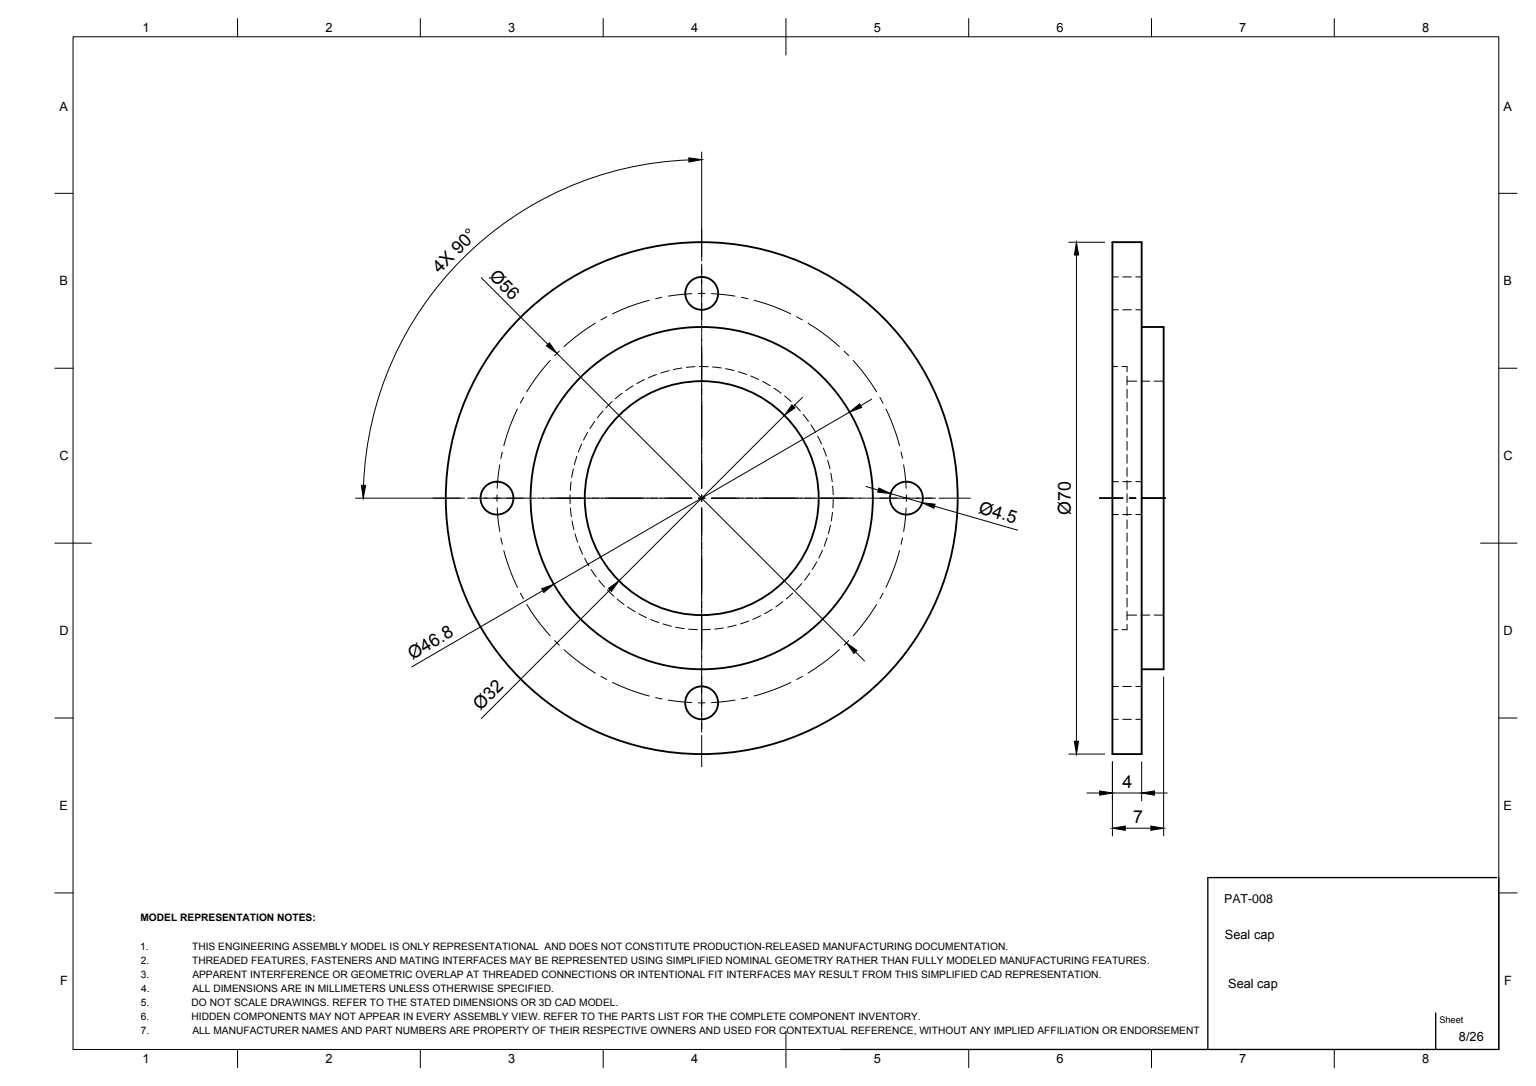
ISO-10303-21;
HEADER;
/* Generated by software containing ST-Developer
 * from STEP Tools, Inc. (www.steptools.com) 
 */

FILE_DESCRIPTION(
/* description */ ('Bearing housing with oil seal and end cap'),
/* implementation_level */ '2;1');

FILE_NAME(
/* name */ 'Seal cap.step',
/* time_stamp */ '2026-10-28T03:23:10-07:00',
/* author */ (''),
/* organization */ (''),
/* preprocessor_version */ 'ST-DEVELOPER v20.2',
/* originating_system */ 'Autodesk Translation Framework v15.17.0.0',
/* authorisation */ '');

FILE_SCHEMA (('AUTOMOTIVE_DESIGN { 1 0 10303 214 3 1 1 }'));
ENDSEC;

DATA;
#10=MECHANICAL_DESIGN_GEOMETRIC_PRESENTATION_REPRESENTATION('',(#262),#7871);
#220=SHAPE_REPRESENTATION_RELATIONSHIP('SRR','None',#7967,#241);
#241=ADVANCED_BREP_SHAPE_REPRESENTATION('',(#291),#7851);
#262=STYLED_ITEM('',(#8160),#291);
#291=MANIFOLD_SOLID_BREP('Body1',#4088);
#345=FACE_BOUND('',#895,.T.);
#346=FACE_BOUND('',#898,.T.);
#347=FACE_BOUND('',#902,.T.);
#348=FACE_BOUND('',#903,.T.);
#349=FACE_BOUND('',#904,.T.);
#350=FACE_BOUND('',#905,.T.);
#351=FACE_BOUND('',#906,.T.);
#352=FACE_BOUND('',#908,.T.);
#353=FACE_BOUND('',#909,.T.);
#354=FACE_BOUND('',#910,.T.);
#355=FACE_BOUND('',#911,.T.);
#356=FACE_BOUND('',#912,.T.);
#444=PLANE('',#4473);
#445=PLANE('',#4478);
#446=PLANE('',#4484);
#447=PLANE('',#4485);
#608=FACE_OUTER_BOUND('',#889,.T.);
#609=FACE_OUTER_BOUND('',#890,.T.);
#610=FACE_OUTER_BOUND('',#891,.T.);
#611=FACE_OUTER_BOUND('',#892,.T.);
#612=FACE_OUTER_BOUND('',#893,.T.);
#613=FACE_OUTER_BOUND('',#894,.T.);
#614=FACE_OUTER_BOUND('',#896,.T.);
#615=FACE_OUTER_BOUND('',#897,.T.);
#616=FACE_OUTER_BOUND('',#899,.T.);
#617=FACE_OUTER_BOUND('',#900,.T.);
#618=FACE_OUTER_BOUND('',#901,.T.);
#619=FACE_OUTER_BOUND('',#907,.T.);
#889=EDGE_LOOP('',(#2975,#2976,#2977,#2978));
#890=EDGE_LOOP('',(#2979,#2980,#2981,#2982));
#891=EDGE_LOOP('',(#2983,#2984,#2985,#2986));
#892=EDGE_LOOP('',(#2987,#2988,#2989,#2990));
#893=EDGE_LOOP('',(#2991,#2992,#2993,#2994));
#894=EDGE_LOOP('',(#2995));
#895=EDGE_LOOP('',(#2996));
#896=EDGE_LOOP('',(#2997,#2998,#2999,#3000));
#897=EDGE_LOOP('',(#3001));
#898=EDGE_LOOP('',(#3002));
#899=EDGE_LOOP('',(#3003,#3004,#3005,#3006));
#900=EDGE_LOOP('',(#3007,#3008,#3009,#3010));
#901=EDGE_LOOP('',(#3011));
#902=EDGE_LOOP('',(#3012));
#903=EDGE_LOOP('',(#3013));
#904=EDGE_LOOP('',(#3014));
#905=EDGE_LOOP('',(#3015));
#906=EDGE_LOOP('',(#3016));
#907=EDGE_LOOP('',(#3017));
#908=EDGE_LOOP('',(#3018));
#909=EDGE_LOOP('',(#3019));
#910=EDGE_LOOP('',(#3020));
#911=EDGE_LOOP('',(#3021));
#912=EDGE_LOOP('',(#3022));
#1215=LINE('',#6464,#1477);
#1216=LINE('',#6470,#1478);
#1217=LINE('',#6476,#1479);
#1218=LINE('',#6482,#1480);
#1219=LINE('',#6488,#1481);
#1220=LINE('',#6497,#1482);
#1221=LINE('',#6503,#1483);
#1222=LINE('',#6508,#1484);
#1477=VECTOR('',#5172,0.225);
#1478=VECTOR('',#5179,0.225);
#1479=VECTOR('',#5186,0.225);
#1480=VECTOR('',#5193,0.225);
#1481=VECTOR('',#5200,2.34);
#1482=VECTOR('',#5211,1.8);
#1483=VECTOR('',#5220,1.6);
#1484=VECTOR('',#5225,3.5);
#1719=CIRCLE('',#4459,0.225);
#1720=CIRCLE('',#4460,0.225);
#1721=CIRCLE('',#4462,0.225);
#1722=CIRCLE('',#4463,0.225);
#1723=CIRCLE('',#4465,0.225);
#1724=CIRCLE('',#4466,0.225);
#1725=CIRCLE('',#4468,0.225);
#1726=CIRCLE('',#4469,0.225);
#1727=CIRCLE('',#4471,2.34);
#1728=CIRCLE('',#4472,2.34);
#1729=CIRCLE('',#4474,1.6);
#1730=CIRCLE('',#4476,1.8);
#1731=CIRCLE('',#4477,1.8);
#1732=CIRCLE('',#4479,1.6);
#1733=CIRCLE('',#4482,3.5);
#1734=CIRCLE('',#4483,3.5);
#1967=VERTEX_POINT('',#6461);
#1968=VERTEX_POINT('',#6463);
#1969=VERTEX_POINT('',#6467);
#1970=VERTEX_POINT('',#6469);
#1971=VERTEX_POINT('',#6473);
#1972=VERTEX_POINT('',#6475);
#1973=VERTEX_POINT('',#6479);
#1974=VERTEX_POINT('',#6481);
#1975=VERTEX_POINT('',#6485);
#1976=VERTEX_POINT('',#6487);
#1977=VERTEX_POINT('',#6491);
#1978=VERTEX_POINT('',#6494);
#1979=VERTEX_POINT('',#6496);
#1980=VERTEX_POINT('',#6500);
#1981=VERTEX_POINT('',#6505);
#1982=VERTEX_POINT('',#6507);
#2351=EDGE_CURVE('',#1967,#1967,#1719,.T.);
#2352=EDGE_CURVE('',#1967,#1968,#1215,.T.);
#2353=EDGE_CURVE('',#1968,#1968,#1720,.T.);
#2354=EDGE_CURVE('',#1969,#1969,#1721,.T.);
#2355=EDGE_CURVE('',#1969,#1970,#1216,.T.);
#2356=EDGE_CURVE('',#1970,#1970,#1722,.T.);
#2357=EDGE_CURVE('',#1971,#1971,#1723,.T.);
#2358=EDGE_CURVE('',#1971,#1972,#1217,.T.);
#2359=EDGE_CURVE('',#1972,#1972,#1724,.T.);
#2360=EDGE_CURVE('',#1973,#1973,#1725,.T.);
#2361=EDGE_CURVE('',#1973,#1974,#1218,.T.);
#2362=EDGE_CURVE('',#1974,#1974,#1726,.T.);
#2363=EDGE_CURVE('',#1975,#1975,#1727,.T.);
#2364=EDGE_CURVE('',#1975,#1976,#1219,.T.);
#2365=EDGE_CURVE('',#1976,#1976,#1728,.T.);
#2366=EDGE_CURVE('',#1977,#1977,#1729,.T.);
#2367=EDGE_CURVE('',#1978,#1978,#1730,.T.);
#2368=EDGE_CURVE('',#1978,#1979,#1220,.T.);
#2369=EDGE_CURVE('',#1979,#1979,#1731,.T.);
#2370=EDGE_CURVE('',#1980,#1980,#1732,.T.);
#2371=EDGE_CURVE('',#1977,#1980,#1221,.T.);
#2372=EDGE_CURVE('',#1981,#1981,#1733,.T.);
#2373=EDGE_CURVE('',#1981,#1982,#1222,.T.);
#2374=EDGE_CURVE('',#1982,#1982,#1734,.T.);
#2975=ORIENTED_EDGE('',*,*,#2351,.F.);
#2976=ORIENTED_EDGE('',*,*,#2352,.T.);
#2977=ORIENTED_EDGE('',*,*,#2353,.F.);
#2978=ORIENTED_EDGE('',*,*,#2352,.F.);
#2979=ORIENTED_EDGE('',*,*,#2354,.F.);
#2980=ORIENTED_EDGE('',*,*,#2355,.T.);
#2981=ORIENTED_EDGE('',*,*,#2356,.F.);
#2982=ORIENTED_EDGE('',*,*,#2355,.F.);
#2983=ORIENTED_EDGE('',*,*,#2357,.F.);
#2984=ORIENTED_EDGE('',*,*,#2358,.T.);
#2985=ORIENTED_EDGE('',*,*,#2359,.F.);
#2986=ORIENTED_EDGE('',*,*,#2358,.F.);
#2987=ORIENTED_EDGE('',*,*,#2360,.F.);
#2988=ORIENTED_EDGE('',*,*,#2361,.T.);
#2989=ORIENTED_EDGE('',*,*,#2362,.F.);
#2990=ORIENTED_EDGE('',*,*,#2361,.F.);
#2991=ORIENTED_EDGE('',*,*,#2363,.F.);
#2992=ORIENTED_EDGE('',*,*,#2364,.T.);
#2993=ORIENTED_EDGE('',*,*,#2365,.F.);
#2994=ORIENTED_EDGE('',*,*,#2364,.F.);
#2995=ORIENTED_EDGE('',*,*,#2363,.T.);
#2996=ORIENTED_EDGE('',*,*,#2366,.T.);
#2997=ORIENTED_EDGE('',*,*,#2367,.F.);
#2998=ORIENTED_EDGE('',*,*,#2368,.T.);
#2999=ORIENTED_EDGE('',*,*,#2369,.T.);
#3000=ORIENTED_EDGE('',*,*,#2368,.F.);
#3001=ORIENTED_EDGE('',*,*,#2369,.F.);
#3002=ORIENTED_EDGE('',*,*,#2370,.F.);
#3003=ORIENTED_EDGE('',*,*,#2366,.F.);
#3004=ORIENTED_EDGE('',*,*,#2371,.T.);
#3005=ORIENTED_EDGE('',*,*,#2370,.T.);
#3006=ORIENTED_EDGE('',*,*,#2371,.F.);
#3007=ORIENTED_EDGE('',*,*,#2372,.F.);
#3008=ORIENTED_EDGE('',*,*,#2373,.T.);
#3009=ORIENTED_EDGE('',*,*,#2374,.T.);
#3010=ORIENTED_EDGE('',*,*,#2373,.F.);
#3011=ORIENTED_EDGE('',*,*,#2372,.T.);
#3012=ORIENTED_EDGE('',*,*,#2365,.T.);
#3013=ORIENTED_EDGE('',*,*,#2362,.T.);
#3014=ORIENTED_EDGE('',*,*,#2359,.T.);
#3015=ORIENTED_EDGE('',*,*,#2356,.T.);
#3016=ORIENTED_EDGE('',*,*,#2353,.T.);
#3017=ORIENTED_EDGE('',*,*,#2374,.F.);
#3018=ORIENTED_EDGE('',*,*,#2367,.T.);
#3019=ORIENTED_EDGE('',*,*,#2360,.T.);
#3020=ORIENTED_EDGE('',*,*,#2357,.T.);
#3021=ORIENTED_EDGE('',*,*,#2354,.T.);
#3022=ORIENTED_EDGE('',*,*,#2351,.T.);
#3779=CYLINDRICAL_SURFACE('',#4458,0.225);
#3780=CYLINDRICAL_SURFACE('',#4461,0.225);
#3781=CYLINDRICAL_SURFACE('',#4464,0.225);
#3782=CYLINDRICAL_SURFACE('',#4467,0.225);
#3783=CYLINDRICAL_SURFACE('',#4470,2.34);
#3784=CYLINDRICAL_SURFACE('',#4475,1.8);
#3785=CYLINDRICAL_SURFACE('',#4480,1.6);
#3786=CYLINDRICAL_SURFACE('',#4481,3.5);
#3890=ADVANCED_FACE('',(#608),#3779,.F.);
#3891=ADVANCED_FACE('',(#609),#3780,.F.);
#3892=ADVANCED_FACE('',(#610),#3781,.F.);
#3893=ADVANCED_FACE('',(#611),#3782,.F.);
#3894=ADVANCED_FACE('',(#612),#3783,.T.);
#3895=ADVANCED_FACE('',(#613,#345),#444,.T.);
#3896=ADVANCED_FACE('',(#614),#3784,.F.);
#3897=ADVANCED_FACE('',(#615,#346),#445,.F.);
#3898=ADVANCED_FACE('',(#616),#3785,.F.);
#3899=ADVANCED_FACE('',(#617),#3786,.T.);
#3900=ADVANCED_FACE('',(#618,#347,#348,#349,#350,#351),#446,.T.);
#3901=ADVANCED_FACE('',(#619,#352,#353,#354,#355,#356),#447,.F.);
#4088=CLOSED_SHELL('',(#3890,#3891,#3892,#3893,#3894,#3895,#3896,#3897,
#3898,#3899,#3900,#3901));
#4457=AXIS2_PLACEMENT_3D('',#6459,#5166,#5167);
#4458=AXIS2_PLACEMENT_3D('',#6460,#5168,#5169);
#4459=AXIS2_PLACEMENT_3D('',#6462,#5170,#5171);
#4460=AXIS2_PLACEMENT_3D('',#6465,#5173,#5174);
#4461=AXIS2_PLACEMENT_3D('',#6466,#5175,#5176);
#4462=AXIS2_PLACEMENT_3D('',#6468,#5177,#5178);
#4463=AXIS2_PLACEMENT_3D('',#6471,#5180,#5181);
#4464=AXIS2_PLACEMENT_3D('',#6472,#5182,#5183);
#4465=AXIS2_PLACEMENT_3D('',#6474,#5184,#5185);
#4466=AXIS2_PLACEMENT_3D('',#6477,#5187,#5188);
#4467=AXIS2_PLACEMENT_3D('',#6478,#5189,#5190);
#4468=AXIS2_PLACEMENT_3D('',#6480,#5191,#5192);
#4469=AXIS2_PLACEMENT_3D('',#6483,#5194,#5195);
#4470=AXIS2_PLACEMENT_3D('',#6484,#5196,#5197);
#4471=AXIS2_PLACEMENT_3D('',#6486,#5198,#5199);
#4472=AXIS2_PLACEMENT_3D('',#6489,#5201,#5202);
#4473=AXIS2_PLACEMENT_3D('',#6490,#5203,#5204);
#4474=AXIS2_PLACEMENT_3D('',#6492,#5205,#5206);
#4475=AXIS2_PLACEMENT_3D('',#6493,#5207,#5208);
#4476=AXIS2_PLACEMENT_3D('',#6495,#5209,#5210);
#4477=AXIS2_PLACEMENT_3D('',#6498,#5212,#5213);
#4478=AXIS2_PLACEMENT_3D('',#6499,#5214,#5215);
#4479=AXIS2_PLACEMENT_3D('',#6501,#5216,#5217);
#4480=AXIS2_PLACEMENT_3D('',#6502,#5218,#5219);
#4481=AXIS2_PLACEMENT_3D('',#6504,#5221,#5222);
#4482=AXIS2_PLACEMENT_3D('',#6506,#5223,#5224);
#4483=AXIS2_PLACEMENT_3D('',#6509,#5226,#5227);
#4484=AXIS2_PLACEMENT_3D('',#6510,#5228,#5229);
#4485=AXIS2_PLACEMENT_3D('',#6511,#5230,#5231);
#5166=DIRECTION('axis',(0.,0.,1.));
#5167=DIRECTION('refdir',(1.,0.,0.));
#5168=DIRECTION('center_axis',(0.,1.,0.));
#5169=DIRECTION('ref_axis',(1.,0.,0.));
#5170=DIRECTION('center_axis',(0.,1.,0.));
#5171=DIRECTION('ref_axis',(1.,0.,0.));
#5172=DIRECTION('',(0.,1.,0.));
#5173=DIRECTION('center_axis',(0.,-1.,0.));
#5174=DIRECTION('ref_axis',(1.,0.,0.));
#5175=DIRECTION('center_axis',(0.,1.,0.));
#5176=DIRECTION('ref_axis',(1.,0.,0.));
#5177=DIRECTION('center_axis',(0.,1.,0.));
#5178=DIRECTION('ref_axis',(1.,0.,0.));
#5179=DIRECTION('',(0.,1.,0.));
#5180=DIRECTION('center_axis',(0.,-1.,0.));
#5181=DIRECTION('ref_axis',(1.,0.,0.));
#5182=DIRECTION('center_axis',(0.,1.,0.));
#5183=DIRECTION('ref_axis',(1.,0.,0.));
#5184=DIRECTION('center_axis',(0.,1.,0.));
#5185=DIRECTION('ref_axis',(1.,0.,0.));
#5186=DIRECTION('',(0.,1.,0.));
#5187=DIRECTION('center_axis',(0.,-1.,0.));
#5188=DIRECTION('ref_axis',(1.,0.,0.));
#5189=DIRECTION('center_axis',(0.,1.,0.));
#5190=DIRECTION('ref_axis',(1.,0.,0.));
#5191=DIRECTION('center_axis',(0.,1.,0.));
#5192=DIRECTION('ref_axis',(1.,0.,0.));
#5193=DIRECTION('',(0.,1.,0.));
#5194=DIRECTION('center_axis',(0.,-1.,0.));
#5195=DIRECTION('ref_axis',(1.,0.,0.));
#5196=DIRECTION('center_axis',(0.,1.,0.));
#5197=DIRECTION('ref_axis',(1.,0.,0.));
#5198=DIRECTION('center_axis',(0.,1.,0.));
#5199=DIRECTION('ref_axis',(1.,0.,0.));
#5200=DIRECTION('',(0.,-1.,0.));
#5201=DIRECTION('center_axis',(0.,-1.,0.));
#5202=DIRECTION('ref_axis',(1.,0.,0.));
#5203=DIRECTION('center_axis',(0.,1.,0.));
#5204=DIRECTION('ref_axis',(1.,0.,0.));
#5205=DIRECTION('center_axis',(0.,-1.,0.));
#5206=DIRECTION('ref_axis',(1.,0.,0.));
#5207=DIRECTION('center_axis',(0.,1.,0.));
#5208=DIRECTION('ref_axis',(1.,0.,0.));
#5209=DIRECTION('center_axis',(0.,1.,0.));
#5210=DIRECTION('ref_axis',(1.,0.,0.));
#5211=DIRECTION('',(0.,1.,0.));
#5212=DIRECTION('center_axis',(0.,1.,0.));
#5213=DIRECTION('ref_axis',(1.,0.,0.));
#5214=DIRECTION('center_axis',(0.,1.,0.));
#5215=DIRECTION('ref_axis',(1.,0.,0.));
#5216=DIRECTION('center_axis',(0.,-1.,0.));
#5217=DIRECTION('ref_axis',(1.,0.,0.));
#5218=DIRECTION('center_axis',(0.,1.,0.));
#5219=DIRECTION('ref_axis',(1.,0.,0.));
#5220=DIRECTION('',(0.,-1.,0.));
#5221=DIRECTION('center_axis',(0.,1.,0.));
#5222=DIRECTION('ref_axis',(1.,0.,0.));
#5223=DIRECTION('center_axis',(0.,1.,0.));
#5224=DIRECTION('ref_axis',(1.,0.,0.));
#5225=DIRECTION('',(0.,-1.,0.));
#5226=DIRECTION('center_axis',(0.,1.,0.));
#5227=DIRECTION('ref_axis',(1.,0.,0.));
#5228=DIRECTION('center_axis',(0.,1.,0.));
#5229=DIRECTION('ref_axis',(1.,0.,0.));
#5230=DIRECTION('center_axis',(0.,1.,0.));
#5231=DIRECTION('ref_axis',(1.,0.,0.));
#6459=CARTESIAN_POINT('',(0.,0.,0.));
#6460=CARTESIAN_POINT('Origin',(-2.8,-0.5,4.5));
#6461=CARTESIAN_POINT('',(-3.025,-0.4,4.5));
#6462=CARTESIAN_POINT('Origin',(-2.8,-0.4,4.5));
#6463=CARTESIAN_POINT('',(-3.025,0.,4.5));
#6464=CARTESIAN_POINT('',(-3.025,-0.5,4.5));
#6465=CARTESIAN_POINT('Origin',(-2.8,0.,4.5));
#6466=CARTESIAN_POINT('Origin',(1.71450551880629E-16,-0.5,7.3));
#6467=CARTESIAN_POINT('',(-0.225,-0.4,7.3));
#6468=CARTESIAN_POINT('Origin',(1.71450551880629E-16,-0.4,7.3));
#6469=CARTESIAN_POINT('',(-0.225,0.,7.3));
#6470=CARTESIAN_POINT('',(-0.225,-0.5,7.3));
#6471=CARTESIAN_POINT('Origin',(1.71450551880629E-16,0.,7.3));
#6472=CARTESIAN_POINT('Origin',(2.8,-0.5,4.5));
#6473=CARTESIAN_POINT('',(2.575,-0.4,4.5));
#6474=CARTESIAN_POINT('Origin',(2.8,-0.4,4.5));
#6475=CARTESIAN_POINT('',(2.575,0.,4.5));
#6476=CARTESIAN_POINT('',(2.575,-0.5,4.5));
#6477=CARTESIAN_POINT('Origin',(2.8,0.,4.5));
#6478=CARTESIAN_POINT('Origin',(-5.14351655641888E-16,-0.5,1.7));
#6479=CARTESIAN_POINT('',(-0.225000000000001,-0.4,1.7));
#6480=CARTESIAN_POINT('Origin',(-5.14351655641888E-16,-0.4,1.7));
#6481=CARTESIAN_POINT('',(-0.225000000000001,0.,1.7));
#6482=CARTESIAN_POINT('',(-0.225000000000001,-0.5,1.7));
#6483=CARTESIAN_POINT('Origin',(-5.14351655641888E-16,0.,1.7));
#6484=CARTESIAN_POINT('Origin',(0.,0.,4.5));
#6485=CARTESIAN_POINT('',(-2.34,0.3,4.5));
#6486=CARTESIAN_POINT('Origin',(0.,0.3,4.5));
#6487=CARTESIAN_POINT('',(-2.34,0.,4.5));
#6488=CARTESIAN_POINT('',(-2.34,0.,4.5));
#6489=CARTESIAN_POINT('Origin',(0.,0.,4.5));
#6490=CARTESIAN_POINT('Origin',(0.,0.3,4.5));
#6491=CARTESIAN_POINT('',(-1.6,0.3,4.5));
#6492=CARTESIAN_POINT('Origin',(0.,0.3,4.5));
#6493=CARTESIAN_POINT('Origin',(0.,-0.41,4.5));
#6494=CARTESIAN_POINT('',(-1.8,-0.4,4.5));
#6495=CARTESIAN_POINT('Origin',(0.,-0.4,4.5));
#6496=CARTESIAN_POINT('',(-1.8,-0.2,4.5));
#6497=CARTESIAN_POINT('',(-1.8,-0.41,4.5));
#6498=CARTESIAN_POINT('Origin',(0.,-0.2,4.5));
#6499=CARTESIAN_POINT('Origin',(0.,-0.2,4.5));
#6500=CARTESIAN_POINT('',(-1.6,-0.2,4.5));
#6501=CARTESIAN_POINT('Origin',(0.,-0.2,4.5));
#6502=CARTESIAN_POINT('Origin',(0.,-0.4,4.5));
#6503=CARTESIAN_POINT('',(-1.6,-0.4,4.5));
#6504=CARTESIAN_POINT('Origin',(0.,-0.4,4.5));
#6505=CARTESIAN_POINT('',(-3.5,0.,4.5));
#6506=CARTESIAN_POINT('Origin',(0.,0.,4.5));
#6507=CARTESIAN_POINT('',(-3.5,-0.4,4.5));
#6508=CARTESIAN_POINT('',(-3.5,-0.4,4.5));
#6509=CARTESIAN_POINT('Origin',(0.,-0.4,4.5));
#6510=CARTESIAN_POINT('Origin',(0.,0.,4.5));
#6511=CARTESIAN_POINT('Origin',(0.,-0.4,4.5));
#7825=UNCERTAINTY_MEASURE_WITH_UNIT(LENGTH_MEASURE(0.001),#7872,
'DISTANCE_ACCURACY_VALUE',
'Maximum model space distance between geometric entities at asserted c
onnectivities');
#7845=UNCERTAINTY_MEASURE_WITH_UNIT(LENGTH_MEASURE(0.001),#7872,
'DISTANCE_ACCURACY_VALUE',
'Maximum model space distance between geometric entities at asserted c
onnectivities');
#7851=(
GEOMETRIC_REPRESENTATION_CONTEXT(3)
GLOBAL_UNCERTAINTY_ASSIGNED_CONTEXT((#7825))
GLOBAL_UNIT_ASSIGNED_CONTEXT((#7872,#7874,#7875))
REPRESENTATION_CONTEXT('','3D')
);
#7871=(
GEOMETRIC_REPRESENTATION_CONTEXT(3)
GLOBAL_UNCERTAINTY_ASSIGNED_CONTEXT((#7845))
GLOBAL_UNIT_ASSIGNED_CONTEXT((#7872,#7874,#7875))
REPRESENTATION_CONTEXT('','3D')
);
#7872=(
LENGTH_UNIT()
NAMED_UNIT(*)
SI_UNIT(.CENTI.,.METRE.)
);
#7874=(
NAMED_UNIT(*)
PLANE_ANGLE_UNIT()
SI_UNIT($,.RADIAN.)
);
#7875=(
NAMED_UNIT(*)
SI_UNIT($,.STERADIAN.)
SOLID_ANGLE_UNIT()
);
#7881=SHAPE_DEFINITION_REPRESENTATION(#7906,#7967);
#7906=PRODUCT_DEFINITION_SHAPE('',$,#7993);
#7967=SHAPE_REPRESENTATION('',(#4457),#7851);
#7987=PRODUCT_DEFINITION_CONTEXT('part definition',#8064,'design');
#7993=PRODUCT_DEFINITION('Seal cap','Seal cap',#8018,#7987);
#8018=PRODUCT_DEFINITION_FORMATION('',$,#8071);
#8064=APPLICATION_CONTEXT(
'Core Data for Automotive Mechanical Design Process');
#8065=PRODUCT_CONTEXT('part definition',#8064,'mechanical');
#8071=PRODUCT('Seal cap','Seal cap','Seal cap',(#8065));
#8154=COLOUR_RGB('Black',0.12,0.14,0.17);
#8155=FILL_AREA_STYLE_COLOUR('',#8154);
#8156=FILL_AREA_STYLE('',(#8155));
#8157=SURFACE_STYLE_FILL_AREA(#8156);
#8158=SURFACE_SIDE_STYLE('',(#8157));
#8159=SURFACE_STYLE_USAGE(.BOTH.,#8158);
#8160=PRESENTATION_STYLE_ASSIGNMENT((#8159));
ENDSEC;
END-ISO-10303-21;
